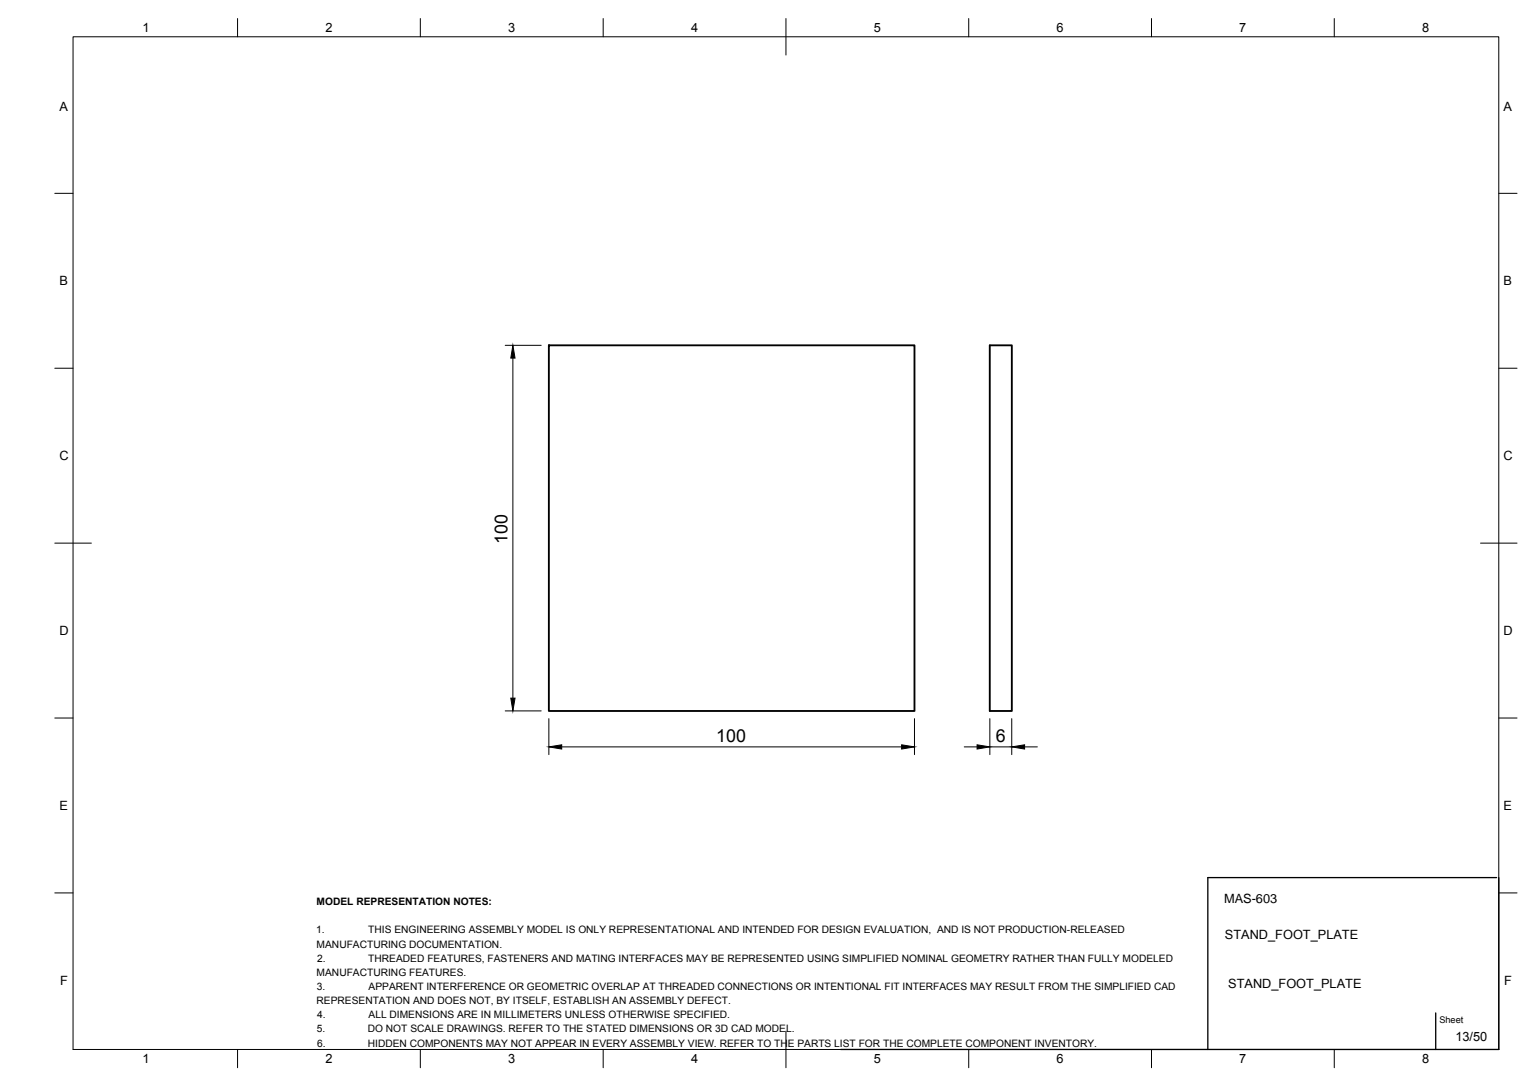
ISO-10303-21;
HEADER;
FILE_DESCRIPTION((''),'2;1');
FILE_NAME('STAND_FOOT_PLATE.step','2026-10-01T22:06:14-07:00',(''),(''),'','','');
FILE_SCHEMA (('AUTOMOTIVE_DESIGN { 1 0 10303 214 3 1 1 }'));
ENDSEC;
DATA;
#10=MECHANICAL_DESIGN_GEOMETRIC_PRESENTATION_REPRESENTATION('',(#987),#50440);
#897=SHAPE_REPRESENTATION_RELATIONSHIP('SRR','None',#50628,#942) ;
#942=ADVANCED_BREP_SHAPE_REPRESENTATION('',(#1042),#50397) ;
#987=STYLED_ITEM('',(#50883),#1042) ;
#1042=MANIFOLD_SOLID_BREP('STAND_FOOT_PLATE',#28654) ;
#1920=PLANE('',#30247) ;
#1921=PLANE('',#30248) ;
#1922=PLANE('',#30249) ;
#1923=PLANE('',#30250) ;
#1924=PLANE('',#30251) ;
#1925=PLANE('',#30252) ;
#3007=FACE_OUTER_BOUND('',#4719,.T.) ;
#3008=FACE_OUTER_BOUND('',#4720,.T.) ;
#3009=FACE_OUTER_BOUND('',#4721,.T.) ;
#3010=FACE_OUTER_BOUND('',#4722,.T.) ;
#3011=FACE_OUTER_BOUND('',#4723,.T.) ;
#3012=FACE_OUTER_BOUND('',#4724,.T.) ;
#4719=EDGE_LOOP('',(#22087,#22088,#22089,#22090)) ;
#4720=EDGE_LOOP('',(#22091,#22092,#22093,#22094)) ;
#4721=EDGE_LOOP('',(#22095,#22096,#22097,#22098)) ;
#4722=EDGE_LOOP('',(#22099,#22100,#22101,#22102)) ;
#4723=EDGE_LOOP('',(#22103,#22104,#22105,#22106)) ;
#4724=EDGE_LOOP('',(#22107,#22108,#22109,#22110)) ;
#7123=LINE('',#44846,#9595) ;
#7124=LINE('',#44848,#9596) ;
#7125=LINE('',#44850,#9597) ;
#7126=LINE('',#44851,#9598) ;
#7127=LINE('',#44855,#9599) ;
#7128=LINE('',#44857,#9600) ;
#7129=LINE('',#44859,#9601) ;
#7130=LINE('',#44860,#9602) ;
#7131=LINE('',#44862,#9603) ;
#7132=LINE('',#44863,#9604) ;
#7133=LINE('',#44865,#9605) ;
#7134=LINE('',#44867,#9606) ;
#9595=VECTOR('',#35844,1.) ;
#9596=VECTOR('',#35845,1.) ;
#9597=VECTOR('',#35846,1.) ;
#9598=VECTOR('',#35847,1.) ;
#9599=VECTOR('',#35850,1.) ;
#9600=VECTOR('',#35851,1.) ;
#9601=VECTOR('',#35852,1.) ;
#9602=VECTOR('',#35853,1.) ;
#9603=VECTOR('',#35856,1.) ;
#9604=VECTOR('',#35857,1.) ;
#9605=VECTOR('',#35860,1.) ;
#9606=VECTOR('',#35863,1.) ;
#13012=VERTEX_POINT('',#44844) ;
#13013=VERTEX_POINT('',#44845) ;
#13014=VERTEX_POINT('',#44847) ;
#13015=VERTEX_POINT('',#44849) ;
#13016=VERTEX_POINT('',#44853) ;
#13017=VERTEX_POINT('',#44854) ;
#13018=VERTEX_POINT('',#44856) ;
#13019=VERTEX_POINT('',#44858) ;
#16309=EDGE_CURVE('',#13012,#13013,#7123,.T.) ;
#16310=EDGE_CURVE('',#13013,#13014,#7124,.T.) ;
#16311=EDGE_CURVE('',#13014,#13015,#7125,.T.) ;
#16312=EDGE_CURVE('',#13015,#13012,#7126,.T.) ;
#16313=EDGE_CURVE('',#13016,#13017,#7127,.T.) ;
#16314=EDGE_CURVE('',#13017,#13018,#7128,.T.) ;
#16315=EDGE_CURVE('',#13018,#13019,#7129,.T.) ;
#16316=EDGE_CURVE('',#13019,#13016,#7130,.T.) ;
#16317=EDGE_CURVE('',#13015,#13018,#7131,.T.) ;
#16318=EDGE_CURVE('',#13012,#13017,#7132,.T.) ;
#16319=EDGE_CURVE('',#13014,#13019,#7133,.T.) ;
#16320=EDGE_CURVE('',#13013,#13016,#7134,.T.) ;
#22087=ORIENTED_EDGE('',*,*,#16309,.T.) ;
#22088=ORIENTED_EDGE('',*,*,#16310,.T.) ;
#22089=ORIENTED_EDGE('',*,*,#16311,.T.) ;
#22090=ORIENTED_EDGE('',*,*,#16312,.T.) ;
#22091=ORIENTED_EDGE('',*,*,#16313,.T.) ;
#22092=ORIENTED_EDGE('',*,*,#16314,.T.) ;
#22093=ORIENTED_EDGE('',*,*,#16315,.T.) ;
#22094=ORIENTED_EDGE('',*,*,#16316,.T.) ;
#22095=ORIENTED_EDGE('',*,*,#16317,.T.) ;
#22096=ORIENTED_EDGE('',*,*,#16314,.F.) ;
#22097=ORIENTED_EDGE('',*,*,#16318,.F.) ;
#22098=ORIENTED_EDGE('',*,*,#16312,.F.) ;
#22099=ORIENTED_EDGE('',*,*,#16319,.T.) ;
#22100=ORIENTED_EDGE('',*,*,#16315,.F.) ;
#22101=ORIENTED_EDGE('',*,*,#16317,.F.) ;
#22102=ORIENTED_EDGE('',*,*,#16311,.F.) ;
#22103=ORIENTED_EDGE('',*,*,#16320,.T.) ;
#22104=ORIENTED_EDGE('',*,*,#16316,.F.) ;
#22105=ORIENTED_EDGE('',*,*,#16319,.F.) ;
#22106=ORIENTED_EDGE('',*,*,#16310,.F.) ;
#22107=ORIENTED_EDGE('',*,*,#16318,.T.) ;
#22108=ORIENTED_EDGE('',*,*,#16313,.F.) ;
#22109=ORIENTED_EDGE('',*,*,#16320,.F.) ;
#22110=ORIENTED_EDGE('',*,*,#16309,.F.) ;
#27742=ADVANCED_FACE('',(#3007),#1920,.T.) ;
#27743=ADVANCED_FACE('',(#3008),#1921,.F.) ;
#27744=ADVANCED_FACE('',(#3009),#1922,.F.) ;
#27745=ADVANCED_FACE('',(#3010),#1923,.F.) ;
#27746=ADVANCED_FACE('',(#3011),#1924,.F.) ;
#27747=ADVANCED_FACE('',(#3012),#1925,.F.) ;
#28654=CLOSED_SHELL('',(#27742,#27743,#27744,#27745,#27746,#27747)) ;
#30246=AXIS2_PLACEMENT_3D('',#44842,#35840,#35841) ;
#30247=AXIS2_PLACEMENT_3D('',#44843,#35842,#35843) ;
#30248=AXIS2_PLACEMENT_3D('',#44852,#35848,#35849) ;
#30249=AXIS2_PLACEMENT_3D('',#44861,#35854,#35855) ;
#30250=AXIS2_PLACEMENT_3D('',#44864,#35858,#35859) ;
#30251=AXIS2_PLACEMENT_3D('',#44866,#35861,#35862) ;
#30252=AXIS2_PLACEMENT_3D('',#44868,#35864,#35865) ;
#35840=DIRECTION('axis',(0.,0.,1.)) ;
#35841=DIRECTION('refdir',(1.,0.,0.)) ;
#35842=DIRECTION('center_axis',(0.,0.,1.)) ;
#35843=DIRECTION('ref_axis',(1.,0.,0.)) ;
#35844=DIRECTION('',(0.,1.,0.)) ;
#35845=DIRECTION('',(-1.,0.,0.)) ;
#35846=DIRECTION('',(0.,-1.,0.)) ;
#35847=DIRECTION('',(1.,0.,0.)) ;
#35848=DIRECTION('center_axis',(0.,0.,1.)) ;
#35849=DIRECTION('ref_axis',(1.,0.,0.)) ;
#35850=DIRECTION('',(0.,-1.,0.)) ;
#35851=DIRECTION('',(-1.,0.,0.)) ;
#35852=DIRECTION('',(0.,1.,0.)) ;
#35853=DIRECTION('',(1.,0.,0.)) ;
#35854=DIRECTION('center_axis',(0.,1.,0.)) ;
#35855=DIRECTION('ref_axis',(0.,0.,1.)) ;
#35856=DIRECTION('',(0.,0.,-1.)) ;
#35857=DIRECTION('',(0.,0.,-1.)) ;
#35858=DIRECTION('center_axis',(1.,0.,0.)) ;
#35859=DIRECTION('ref_axis',(0.,0.,-1.)) ;
#35860=DIRECTION('',(0.,0.,-1.)) ;
#35861=DIRECTION('center_axis',(0.,-1.,0.)) ;
#35862=DIRECTION('ref_axis',(0.,0.,-1.)) ;
#35863=DIRECTION('',(0.,0.,-1.)) ;
#35864=DIRECTION('center_axis',(-1.,0.,0.)) ;
#35865=DIRECTION('ref_axis',(0.,0.,1.)) ;
#44842=CARTESIAN_POINT('',(0.,0.,0.)) ;
#44843=CARTESIAN_POINT('Origin',(0.,0.,0.6)) ;
#44844=CARTESIAN_POINT('',(5.,-5.,0.6)) ;
#44845=CARTESIAN_POINT('',(5.,5.,0.6)) ;
#44846=CARTESIAN_POINT('',(5.,0.,0.6)) ;
#44847=CARTESIAN_POINT('',(-5.,5.,0.6)) ;
#44848=CARTESIAN_POINT('',(0.,5.,0.6)) ;
#44849=CARTESIAN_POINT('',(-5.,-5.,0.6)) ;
#44850=CARTESIAN_POINT('',(-5.,0.,0.6)) ;
#44851=CARTESIAN_POINT('',(0.,-5.,0.6)) ;
#44852=CARTESIAN_POINT('Origin',(0.,0.,0.)) ;
#44853=CARTESIAN_POINT('',(5.,5.,0.)) ;
#44854=CARTESIAN_POINT('',(5.,-5.,0.)) ;
#44855=CARTESIAN_POINT('',(5.,0.,0.)) ;
#44856=CARTESIAN_POINT('',(-5.,-5.,0.)) ;
#44857=CARTESIAN_POINT('',(0.,-5.,0.)) ;
#44858=CARTESIAN_POINT('',(-5.,5.,0.)) ;
#44859=CARTESIAN_POINT('',(-5.,0.,0.)) ;
#44860=CARTESIAN_POINT('',(0.,5.,0.)) ;
#44861=CARTESIAN_POINT('Origin',(0.,-5.,0.3)) ;
#44862=CARTESIAN_POINT('',(-5.,-5.,0.3)) ;
#44863=CARTESIAN_POINT('',(5.,-5.,0.3)) ;
#44864=CARTESIAN_POINT('Origin',(-5.,0.,0.3)) ;
#44865=CARTESIAN_POINT('',(-5.,5.,0.3)) ;
#44866=CARTESIAN_POINT('Origin',(0.,5.,0.3)) ;
#44867=CARTESIAN_POINT('',(5.,5.,0.3)) ;
#44868=CARTESIAN_POINT('Origin',(5.,0.,0.3)) ;
#50344=UNCERTAINTY_MEASURE_WITH_UNIT(LENGTH_MEASURE(0.001),#50441,
'DISTANCE_ACCURACY_VALUE',
'Maximum model space distance between geometric entities at asserted c
onnectivities') ;
#50387=UNCERTAINTY_MEASURE_WITH_UNIT(LENGTH_MEASURE(0.001),#50441,
'DISTANCE_ACCURACY_VALUE',
'Maximum model space distance between geometric entities at asserted c
onnectivities') ;
#50397=(
GEOMETRIC_REPRESENTATION_CONTEXT(3)
GLOBAL_UNCERTAINTY_ASSIGNED_CONTEXT((#50344))
GLOBAL_UNIT_ASSIGNED_CONTEXT((#50441,#50443,#50444))
REPRESENTATION_CONTEXT('','3D')
) ;
#50440=(
GEOMETRIC_REPRESENTATION_CONTEXT(3)
GLOBAL_UNCERTAINTY_ASSIGNED_CONTEXT((#50387))
GLOBAL_UNIT_ASSIGNED_CONTEXT((#50441,#50443,#50444))
REPRESENTATION_CONTEXT('','3D')
) ;
#50441=(
LENGTH_UNIT()
NAMED_UNIT(*)
SI_UNIT(.CENTI.,.METRE.)
) ;
#50443=(
NAMED_UNIT(*)
PLANE_ANGLE_UNIT()
SI_UNIT($,.RADIAN.)
) ;
#50444=(
NAMED_UNIT(*)
SI_UNIT($,.STERADIAN.)
SOLID_ANGLE_UNIT()
) ;
#50454=SHAPE_DEFINITION_REPRESENTATION(#50512,#50628) ;
#50512=PRODUCT_DEFINITION_SHAPE('',$,#50681) ;
#50628=SHAPE_REPRESENTATION('',(#30246),#50397) ;
#50671=PRODUCT_DEFINITION_CONTEXT('part definition',#50829,'design') ;
#50681=PRODUCT_DEFINITION('STAND_FOOT_PLATE','STAND_FOOT_PLATE',
#50733,#50671) ;
#50733=PRODUCT_DEFINITION_FORMATION('',$,#50840) ;
#50829=APPLICATION_CONTEXT(
'Core Data for Automotive Mechanical Design Process') ;
#50830=PRODUCT_CONTEXT('part definition',#50829,'mechanical') ;
#50840=PRODUCT('STAND_FOOT_PLATE','STAND_FOOT_PLATE',$,(#50830)) ;
#50883=PRESENTATION_STYLE_ASSIGNMENT((#50890)) ;
#50890=SURFACE_STYLE_USAGE(.BOTH.,#50897) ;
#50897=SURFACE_SIDE_STYLE('',(#50904)) ;
#50904=SURFACE_STYLE_FILL_AREA(#50911) ;
#50911=FILL_AREA_STYLE('Steel - Satin',(#50918)) ;
#50918=FILL_AREA_STYLE_COLOUR('Steel - Satin',#50925) ;
#50925=COLOUR_RGB('Steel - Satin', 0.31764706, 0.68627451, 0.89019608) ;
ENDSEC;
END-ISO-10303-21;
